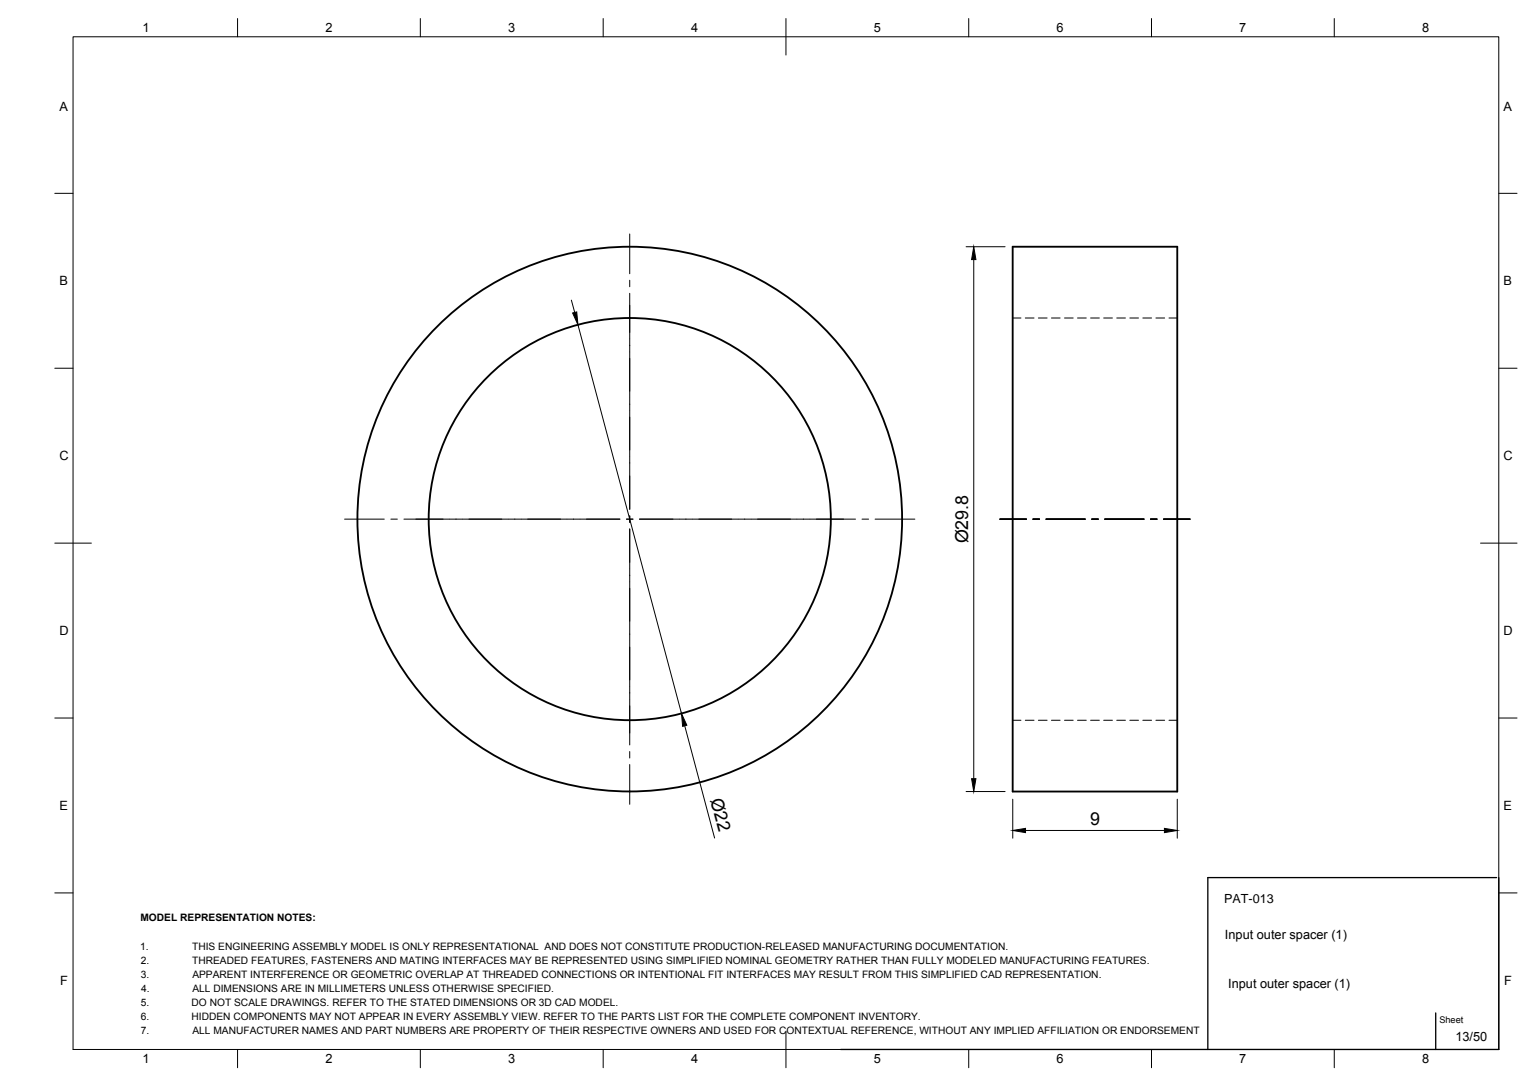
ISO-10303-21;
HEADER;
/* Generated by software containing ST-Developer
 * from STEP Tools, Inc. (www.steptools.com) 
 */

FILE_DESCRIPTION(
/* description */ ('Belt-driven linear axis on 2020 extrusion'),
/* implementation_level */ '2;1');

FILE_NAME(
/* name */ 'Input outer spacer (1).step',
/* time_stamp */ '2026-10-28T03:26:09-07:00',
/* author */ (''),
/* organization */ (''),
/* preprocessor_version */ 'ST-DEVELOPER v20.2',
/* originating_system */ 'Autodesk Translation Framework v15.17.0.0',
/* authorisation */ '');

FILE_SCHEMA (('AUTOMOTIVE_DESIGN { 1 0 10303 214 3 1 1 }'));
ENDSEC;

DATA;
#10=MECHANICAL_DESIGN_GEOMETRIC_PRESENTATION_REPRESENTATION('',(#620),#20096);
#526=SHAPE_REPRESENTATION_RELATIONSHIP('SRR','None',#20322,#572);
#572=ADVANCED_BREP_SHAPE_REPRESENTATION('',(#676),#20053);
#620=STYLED_ITEM('',(#20643),#676);
#676=MANIFOLD_SOLID_BREP('Body1',#10933);
#786=FACE_BOUND('',#2077,.T.);
#787=FACE_BOUND('',#2079,.T.);
#963=PLANE('',#11761);
#964=PLANE('',#11762);
#1384=FACE_OUTER_BOUND('',#2074,.T.);
#1385=FACE_OUTER_BOUND('',#2075,.T.);
#1386=FACE_OUTER_BOUND('',#2076,.T.);
#1387=FACE_OUTER_BOUND('',#2078,.T.);
#2074=EDGE_LOOP('',(#7829,#7830,#7831,#7832));
#2075=EDGE_LOOP('',(#7833,#7834,#7835,#7836));
#2076=EDGE_LOOP('',(#7837));
#2077=EDGE_LOOP('',(#7838));
#2078=EDGE_LOOP('',(#7839));
#2079=EDGE_LOOP('',(#7840));
#2833=LINE('',#16861,#3690);
#2834=LINE('',#16867,#3691);
#3690=VECTOR('',#13487,1.1);
#3691=VECTOR('',#13494,1.49);
#4499=CIRCLE('',#11756,1.1);
#4500=CIRCLE('',#11757,1.1);
#4501=CIRCLE('',#11759,1.49);
#4502=CIRCLE('',#11760,1.49);
#5084=VERTEX_POINT('',#16858);
#5085=VERTEX_POINT('',#16860);
#5086=VERTEX_POINT('',#16864);
#5087=VERTEX_POINT('',#16866);
#6129=EDGE_CURVE('',#5084,#5084,#4499,.T.);
#6130=EDGE_CURVE('',#5084,#5085,#2833,.T.);
#6131=EDGE_CURVE('',#5085,#5085,#4500,.T.);
#6132=EDGE_CURVE('',#5086,#5086,#4501,.T.);
#6133=EDGE_CURVE('',#5086,#5087,#2834,.T.);
#6134=EDGE_CURVE('',#5087,#5087,#4502,.T.);
#7829=ORIENTED_EDGE('',*,*,#6129,.F.);
#7830=ORIENTED_EDGE('',*,*,#6130,.T.);
#7831=ORIENTED_EDGE('',*,*,#6131,.T.);
#7832=ORIENTED_EDGE('',*,*,#6130,.F.);
#7833=ORIENTED_EDGE('',*,*,#6132,.F.);
#7834=ORIENTED_EDGE('',*,*,#6133,.T.);
#7835=ORIENTED_EDGE('',*,*,#6134,.T.);
#7836=ORIENTED_EDGE('',*,*,#6133,.F.);
#7837=ORIENTED_EDGE('',*,*,#6132,.T.);
#7838=ORIENTED_EDGE('',*,*,#6129,.T.);
#7839=ORIENTED_EDGE('',*,*,#6134,.F.);
#7840=ORIENTED_EDGE('',*,*,#6131,.F.);
#10137=CYLINDRICAL_SURFACE('',#11755,1.1);
#10138=CYLINDRICAL_SURFACE('',#11758,1.49);
#10435=ADVANCED_FACE('',(#1384),#10137,.F.);
#10436=ADVANCED_FACE('',(#1385),#10138,.T.);
#10437=ADVANCED_FACE('',(#1386,#786),#963,.T.);
#10438=ADVANCED_FACE('',(#1387,#787),#964,.F.);
#10933=CLOSED_SHELL('',(#10435,#10436,#10437,#10438));
#11754=AXIS2_PLACEMENT_3D('',#16856,#13481,#13482);
#11755=AXIS2_PLACEMENT_3D('',#16857,#13483,#13484);
#11756=AXIS2_PLACEMENT_3D('',#16859,#13485,#13486);
#11757=AXIS2_PLACEMENT_3D('',#16862,#13488,#13489);
#11758=AXIS2_PLACEMENT_3D('',#16863,#13490,#13491);
#11759=AXIS2_PLACEMENT_3D('',#16865,#13492,#13493);
#11760=AXIS2_PLACEMENT_3D('',#16868,#13495,#13496);
#11761=AXIS2_PLACEMENT_3D('',#16869,#13497,#13498);
#11762=AXIS2_PLACEMENT_3D('',#16870,#13499,#13500);
#13481=DIRECTION('axis',(0.,0.,1.));
#13482=DIRECTION('refdir',(1.,0.,0.));
#13483=DIRECTION('center_axis',(0.,1.,0.));
#13484=DIRECTION('ref_axis',(1.,0.,0.));
#13485=DIRECTION('center_axis',(0.,-1.,0.));
#13486=DIRECTION('ref_axis',(1.,0.,0.));
#13487=DIRECTION('',(0.,-1.,0.));
#13488=DIRECTION('center_axis',(0.,-1.,0.));
#13489=DIRECTION('ref_axis',(1.,0.,0.));
#13490=DIRECTION('center_axis',(0.,1.,0.));
#13491=DIRECTION('ref_axis',(1.,0.,0.));
#13492=DIRECTION('center_axis',(0.,1.,0.));
#13493=DIRECTION('ref_axis',(1.,0.,0.));
#13494=DIRECTION('',(0.,-1.,0.));
#13495=DIRECTION('center_axis',(0.,1.,0.));
#13496=DIRECTION('ref_axis',(1.,0.,0.));
#13497=DIRECTION('center_axis',(0.,1.,0.));
#13498=DIRECTION('ref_axis',(1.,0.,0.));
#13499=DIRECTION('center_axis',(0.,1.,0.));
#13500=DIRECTION('ref_axis',(1.,0.,0.));
#16856=CARTESIAN_POINT('',(0.,0.,0.));
#16857=CARTESIAN_POINT('Origin',(32.,-0.45,7.));
#16858=CARTESIAN_POINT('',(30.9,0.45,7.));
#16859=CARTESIAN_POINT('Origin',(32.,0.45,7.));
#16860=CARTESIAN_POINT('',(30.9,-0.45,7.));
#16861=CARTESIAN_POINT('',(30.9,-0.45,7.));
#16862=CARTESIAN_POINT('Origin',(32.,-0.45,7.));
#16863=CARTESIAN_POINT('Origin',(32.,-0.45,7.));
#16864=CARTESIAN_POINT('',(30.51,0.45,7.));
#16865=CARTESIAN_POINT('Origin',(32.,0.45,7.));
#16866=CARTESIAN_POINT('',(30.51,-0.45,7.));
#16867=CARTESIAN_POINT('',(30.51,-0.45,7.));
#16868=CARTESIAN_POINT('Origin',(32.,-0.45,7.));
#16869=CARTESIAN_POINT('Origin',(32.,0.45,7.));
#16870=CARTESIAN_POINT('Origin',(32.,-0.45,7.));
#19999=UNCERTAINTY_MEASURE_WITH_UNIT(LENGTH_MEASURE(0.001),#20097,
'DISTANCE_ACCURACY_VALUE',
'Maximum model space distance between geometric entities at asserted c
onnectivities');
#20042=UNCERTAINTY_MEASURE_WITH_UNIT(LENGTH_MEASURE(0.001),#20097,
'DISTANCE_ACCURACY_VALUE',
'Maximum model space distance between geometric entities at asserted c
onnectivities');
#20053=(
GEOMETRIC_REPRESENTATION_CONTEXT(3)
GLOBAL_UNCERTAINTY_ASSIGNED_CONTEXT((#19999))
GLOBAL_UNIT_ASSIGNED_CONTEXT((#20097,#20099,#20100))
REPRESENTATION_CONTEXT('','3D')
);
#20096=(
GEOMETRIC_REPRESENTATION_CONTEXT(3)
GLOBAL_UNCERTAINTY_ASSIGNED_CONTEXT((#20042))
GLOBAL_UNIT_ASSIGNED_CONTEXT((#20097,#20099,#20100))
REPRESENTATION_CONTEXT('','3D')
);
#20097=(
LENGTH_UNIT()
NAMED_UNIT(*)
SI_UNIT(.CENTI.,.METRE.)
);
#20099=(
NAMED_UNIT(*)
PLANE_ANGLE_UNIT()
SI_UNIT($,.RADIAN.)
);
#20100=(
NAMED_UNIT(*)
SI_UNIT($,.STERADIAN.)
SOLID_ANGLE_UNIT()
);
#20111=SHAPE_DEFINITION_REPRESENTATION(#20164,#20322);
#20164=PRODUCT_DEFINITION_SHAPE('',$,#20376);
#20322=SHAPE_REPRESENTATION('',(#11754),#20053);
#20365=PRODUCT_DEFINITION_CONTEXT('part definition',#20526,'design');
#20376=PRODUCT_DEFINITION('Input outer spacer (1)',
'Input outer spacer (1)',#20429,#20365);
#20429=PRODUCT_DEFINITION_FORMATION('',$,#20538);
#20526=APPLICATION_CONTEXT(
'Core Data for Automotive Mechanical Design Process');
#20527=PRODUCT_CONTEXT('part definition',#20526,'mechanical');
#20538=PRODUCT('Input outer spacer (1)','Input outer spacer (1)',
'Input outer spacer (1)',(#20527));
#20637=COLOUR_RGB('Sky Blue',0.24,0.69,0.87);
#20638=FILL_AREA_STYLE_COLOUR('',#20637);
#20639=FILL_AREA_STYLE('',(#20638));
#20640=SURFACE_STYLE_FILL_AREA(#20639);
#20641=SURFACE_SIDE_STYLE('',(#20640));
#20642=SURFACE_STYLE_USAGE(.BOTH.,#20641);
#20643=PRESENTATION_STYLE_ASSIGNMENT((#20642));
ENDSEC;
END-ISO-10303-21;
